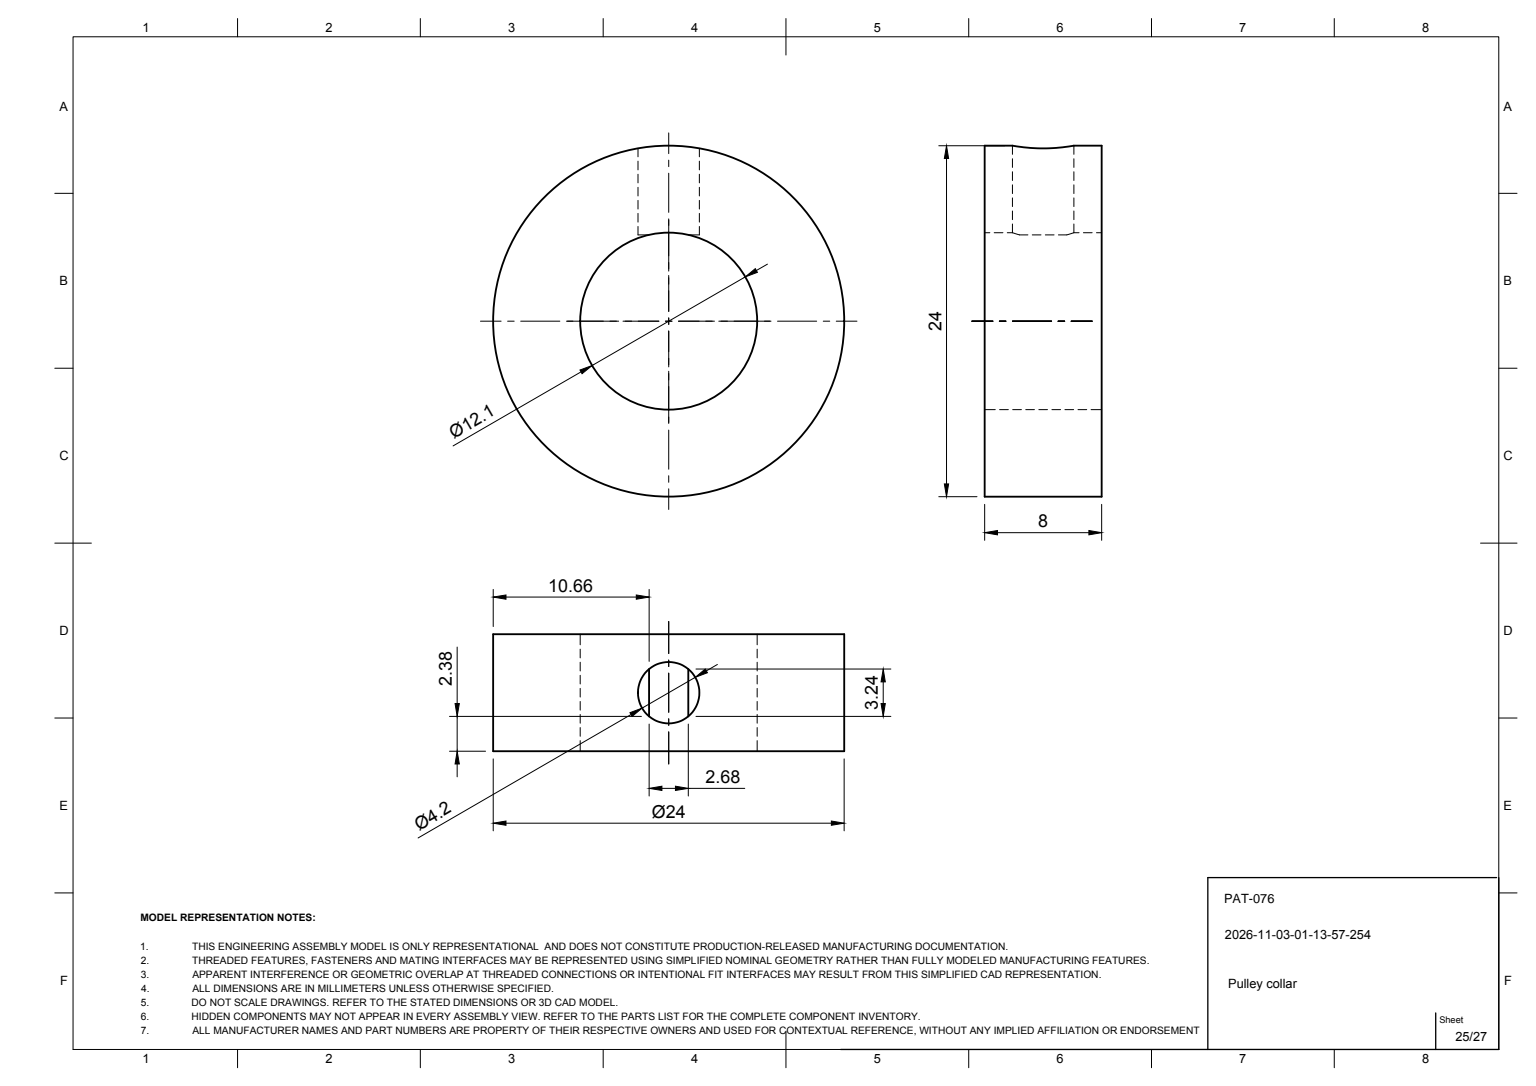
ISO-10303-21;
HEADER;
/* Generated by software containing ST-Developer
 * from STEP Tools, Inc. (www.steptools.com) 
 */

FILE_DESCRIPTION(
/* description */ ('Overhung pulley bearing cartridge'),
/* implementation_level */ '2;1');

FILE_NAME(
/* name */ 'Pulley collar.step',
/* time_stamp */ '2026-10-28T03:22:33-07:00',
/* author */ (''),
/* organization */ (''),
/* preprocessor_version */ 'ST-DEVELOPER v20.2',
/* originating_system */ 'Autodesk Translation Framework v15.17.0.0',
/* authorisation */ '');

FILE_SCHEMA (('AUTOMOTIVE_DESIGN { 1 0 10303 214 3 1 1 }'));
ENDSEC;

DATA;
#10=MECHANICAL_DESIGN_GEOMETRIC_PRESENTATION_REPRESENTATION('',(#309),#10963);
#185=B_SPLINE_CURVE_WITH_KNOTS('',3,(#9899,#9900,#9901,#9902,#9903,#9904,
#9905,#9906,#9907,#9908),.UNSPECIFIED.,.F.,.F.,(4,2,2,2,4),(0.818088904349169,
0.878131747417166,0.957937926194037,1.03774410497091,1.0977869480389),
 .UNSPECIFIED.);
#186=B_SPLINE_CURVE_WITH_KNOTS('',3,(#9914,#9915,#9916,#9917,#9918,#9919,
#9920,#9921,#9922,#9923,#9924,#9925,#9926,#9927,#9928,#9929,#9930,#9931),
 .UNSPECIFIED.,.F.,.F.,(4,2,2,2,2,2,2,2,4),(0.,0.0792812130427884,0.158562426085577,
0.237841058284634,0.317119690483692,0.396398322682749,0.475676954881807,
0.554958167924595,0.634239380967384),.UNSPECIFIED.);
#187=B_SPLINE_CURVE_WITH_KNOTS('',3,(#9932,#9933,#9934,#9935,#9936,#9937,
#9938,#9939,#9940,#9941,#9942,#9943,#9944,#9945,#9946,#9947,#9948,#9949),
 .UNSPECIFIED.,.F.,.F.,(4,2,2,2,2,2,2,2,4),(0.634239380967384,0.713520594010172,
0.792801807052961,0.872080439252018,0.951359071451076,1.03063770365013,
1.10991633584919,1.18919754889198,1.26847876193477),.UNSPECIFIED.);
#188=B_SPLINE_CURVE_WITH_KNOTS('',3,(#9952,#9953,#9954,#9955,#9956,#9957,
#9958,#9959,#9960,#9961),.UNSPECIFIED.,.F.,.F.,(4,2,2,2,4),(0.17946362021981,
0.239506463287808,0.319312642064679,0.39911882084155,0.459161663909547),
 .UNSPECIFIED.);
#257=SHAPE_REPRESENTATION_RELATIONSHIP('SRR','None',#11079,#279);
#279=ADVANCED_BREP_SHAPE_REPRESENTATION('',(#337),#10959);
#309=STYLED_ITEM('',(#11267),#337);
#337=MANIFOLD_SOLID_BREP('Body1',#5678);
#417=FACE_BOUND('',#1190,.T.);
#418=FACE_BOUND('',#1192,.T.);
#419=FACE_BOUND('',#1194,.T.);
#420=FACE_BOUND('',#1196,.T.);
#546=PLANE('',#6370);
#547=PLANE('',#6375);
#548=PLANE('',#6382);
#549=PLANE('',#6383);
#781=FACE_OUTER_BOUND('',#1186,.T.);
#782=FACE_OUTER_BOUND('',#1187,.T.);
#783=FACE_OUTER_BOUND('',#1188,.T.);
#784=FACE_OUTER_BOUND('',#1189,.T.);
#785=FACE_OUTER_BOUND('',#1191,.T.);
#786=FACE_OUTER_BOUND('',#1193,.T.);
#787=FACE_OUTER_BOUND('',#1195,.T.);
#1186=EDGE_LOOP('',(#4467,#4468));
#1187=EDGE_LOOP('',(#4469,#4470,#4471,#4472,#4473,#4474,#4475,#4476,#4477));
#1188=EDGE_LOOP('',(#4478,#4479,#4480));
#1189=EDGE_LOOP('',(#4481,#4482,#4483,#4484));
#1190=EDGE_LOOP('',(#4485,#4486,#4487,#4488));
#1191=EDGE_LOOP('',(#4489,#4490,#4491,#4492));
#1192=EDGE_LOOP('',(#4493,#4494));
#1193=EDGE_LOOP('',(#4495));
#1194=EDGE_LOOP('',(#4496));
#1195=EDGE_LOOP('',(#4497));
#1196=EDGE_LOOP('',(#4498));
#1522=LINE('',#9895,#1864);
#1523=LINE('',#9912,#1865);
#1524=LINE('',#9963,#1866);
#1525=LINE('',#9968,#1867);
#1526=LINE('',#9974,#1868);
#1864=VECTOR('',#7774,1.);
#1865=VECTOR('',#7781,0.21);
#1866=VECTOR('',#7786,1.);
#1867=VECTOR('',#7791,0.605);
#1868=VECTOR('',#7798,1.2);
#2203=CIRCLE('',#6371,0.21);
#2204=CIRCLE('',#6373,0.21);
#2205=CIRCLE('',#6374,0.21);
#2206=CIRCLE('',#6377,0.605);
#2207=CIRCLE('',#6378,0.605);
#2208=CIRCLE('',#6380,1.2);
#2209=CIRCLE('',#6381,1.2);
#2660=VERTEX_POINT('',#9893);
#2661=VERTEX_POINT('',#9894);
#2662=VERTEX_POINT('',#9898);
#2663=VERTEX_POINT('',#9909);
#2664=VERTEX_POINT('',#9911);
#2665=VERTEX_POINT('',#9913);
#2666=VERTEX_POINT('',#9950);
#2667=VERTEX_POINT('',#9965);
#2668=VERTEX_POINT('',#9967);
#2669=VERTEX_POINT('',#9971);
#2670=VERTEX_POINT('',#9973);
#3303=EDGE_CURVE('',#2660,#2661,#1522,.T.);
#3304=EDGE_CURVE('',#2660,#2661,#2203,.T.);
#3305=EDGE_CURVE('',#2662,#2660,#185,.T.);
#3306=EDGE_CURVE('',#2663,#2662,#2204,.T.);
#3307=EDGE_CURVE('',#2663,#2664,#1523,.T.);
#3308=EDGE_CURVE('',#2665,#2664,#186,.T.);
#3309=EDGE_CURVE('',#2664,#2665,#187,.T.);
#3310=EDGE_CURVE('',#2666,#2663,#2205,.T.);
#3311=EDGE_CURVE('',#2661,#2666,#188,.T.);
#3312=EDGE_CURVE('',#2666,#2662,#1524,.T.);
#3313=EDGE_CURVE('',#2667,#2667,#2206,.T.);
#3314=EDGE_CURVE('',#2667,#2668,#1525,.T.);
#3315=EDGE_CURVE('',#2668,#2668,#2207,.T.);
#3316=EDGE_CURVE('',#2669,#2669,#2208,.T.);
#3317=EDGE_CURVE('',#2669,#2670,#1526,.T.);
#3318=EDGE_CURVE('',#2670,#2670,#2209,.T.);
#4467=ORIENTED_EDGE('',*,*,#3303,.F.);
#4468=ORIENTED_EDGE('',*,*,#3304,.T.);
#4469=ORIENTED_EDGE('',*,*,#3305,.F.);
#4470=ORIENTED_EDGE('',*,*,#3306,.F.);
#4471=ORIENTED_EDGE('',*,*,#3307,.T.);
#4472=ORIENTED_EDGE('',*,*,#3308,.F.);
#4473=ORIENTED_EDGE('',*,*,#3309,.F.);
#4474=ORIENTED_EDGE('',*,*,#3307,.F.);
#4475=ORIENTED_EDGE('',*,*,#3310,.F.);
#4476=ORIENTED_EDGE('',*,*,#3311,.F.);
#4477=ORIENTED_EDGE('',*,*,#3304,.F.);
#4478=ORIENTED_EDGE('',*,*,#3312,.F.);
#4479=ORIENTED_EDGE('',*,*,#3310,.T.);
#4480=ORIENTED_EDGE('',*,*,#3306,.T.);
#4481=ORIENTED_EDGE('',*,*,#3313,.F.);
#4482=ORIENTED_EDGE('',*,*,#3314,.T.);
#4483=ORIENTED_EDGE('',*,*,#3315,.T.);
#4484=ORIENTED_EDGE('',*,*,#3314,.F.);
#4485=ORIENTED_EDGE('',*,*,#3311,.T.);
#4486=ORIENTED_EDGE('',*,*,#3312,.T.);
#4487=ORIENTED_EDGE('',*,*,#3305,.T.);
#4488=ORIENTED_EDGE('',*,*,#3303,.T.);
#4489=ORIENTED_EDGE('',*,*,#3316,.F.);
#4490=ORIENTED_EDGE('',*,*,#3317,.T.);
#4491=ORIENTED_EDGE('',*,*,#3318,.T.);
#4492=ORIENTED_EDGE('',*,*,#3317,.F.);
#4493=ORIENTED_EDGE('',*,*,#3308,.T.);
#4494=ORIENTED_EDGE('',*,*,#3309,.T.);
#4495=ORIENTED_EDGE('',*,*,#3316,.T.);
#4496=ORIENTED_EDGE('',*,*,#3313,.T.);
#4497=ORIENTED_EDGE('',*,*,#3318,.F.);
#4498=ORIENTED_EDGE('',*,*,#3315,.F.);
#5229=CYLINDRICAL_SURFACE('',#6372,0.21);
#5230=CYLINDRICAL_SURFACE('',#6376,0.605);
#5231=CYLINDRICAL_SURFACE('',#6379,1.2);
#5525=ADVANCED_FACE('',(#781),#546,.T.);
#5526=ADVANCED_FACE('',(#782),#5229,.F.);
#5527=ADVANCED_FACE('',(#783),#547,.T.);
#5528=ADVANCED_FACE('',(#784,#417),#5230,.F.);
#5529=ADVANCED_FACE('',(#785,#418),#5231,.T.);
#5530=ADVANCED_FACE('',(#786,#419),#548,.T.);
#5531=ADVANCED_FACE('',(#787,#420),#549,.F.);
#5678=CLOSED_SHELL('',(#5525,#5526,#5527,#5528,#5529,#5530,#5531));
#6369=AXIS2_PLACEMENT_3D('',#9891,#7770,#7771);
#6370=AXIS2_PLACEMENT_3D('',#9892,#7772,#7773);
#6371=AXIS2_PLACEMENT_3D('',#9896,#7775,#7776);
#6372=AXIS2_PLACEMENT_3D('',#9897,#7777,#7778);
#6373=AXIS2_PLACEMENT_3D('',#9910,#7779,#7780);
#6374=AXIS2_PLACEMENT_3D('',#9951,#7782,#7783);
#6375=AXIS2_PLACEMENT_3D('',#9962,#7784,#7785);
#6376=AXIS2_PLACEMENT_3D('',#9964,#7787,#7788);
#6377=AXIS2_PLACEMENT_3D('',#9966,#7789,#7790);
#6378=AXIS2_PLACEMENT_3D('',#9969,#7792,#7793);
#6379=AXIS2_PLACEMENT_3D('',#9970,#7794,#7795);
#6380=AXIS2_PLACEMENT_3D('',#9972,#7796,#7797);
#6381=AXIS2_PLACEMENT_3D('',#9975,#7799,#7800);
#6382=AXIS2_PLACEMENT_3D('',#9976,#7801,#7802);
#6383=AXIS2_PLACEMENT_3D('',#9977,#7803,#7804);
#7770=DIRECTION('axis',(0.,0.,1.));
#7771=DIRECTION('refdir',(1.,0.,0.));
#7772=DIRECTION('center_axis',(0.,0.,1.));
#7773=DIRECTION('ref_axis',(1.,0.,0.));
#7774=DIRECTION('',(0.,1.,0.));
#7775=DIRECTION('center_axis',(0.,0.,1.));
#7776=DIRECTION('ref_axis',(1.,0.,0.));
#7777=DIRECTION('center_axis',(0.,0.,1.));
#7778=DIRECTION('ref_axis',(1.,0.,0.));
#7779=DIRECTION('center_axis',(0.,0.,1.));
#7780=DIRECTION('ref_axis',(1.,0.,0.));
#7781=DIRECTION('',(0.,0.,1.));
#7782=DIRECTION('center_axis',(0.,0.,1.));
#7783=DIRECTION('ref_axis',(1.,0.,0.));
#7784=DIRECTION('center_axis',(0.,0.,1.));
#7785=DIRECTION('ref_axis',(1.,0.,0.));
#7786=DIRECTION('',(0.,-1.,0.));
#7787=DIRECTION('center_axis',(0.,1.,0.));
#7788=DIRECTION('ref_axis',(1.,0.,0.));
#7789=DIRECTION('center_axis',(0.,-1.,0.));
#7790=DIRECTION('ref_axis',(1.,0.,0.));
#7791=DIRECTION('',(0.,-1.,0.));
#7792=DIRECTION('center_axis',(0.,-1.,0.));
#7793=DIRECTION('ref_axis',(1.,0.,0.));
#7794=DIRECTION('center_axis',(0.,1.,0.));
#7795=DIRECTION('ref_axis',(1.,0.,0.));
#7796=DIRECTION('center_axis',(0.,1.,0.));
#7797=DIRECTION('ref_axis',(1.,0.,0.));
#7798=DIRECTION('',(0.,-1.,0.));
#7799=DIRECTION('center_axis',(0.,1.,0.));
#7800=DIRECTION('ref_axis',(1.,0.,0.));
#7801=DIRECTION('center_axis',(0.,1.,0.));
#7802=DIRECTION('ref_axis',(1.,0.,0.));
#7803=DIRECTION('center_axis',(0.,1.,0.));
#7804=DIRECTION('ref_axis',(1.,0.,0.));
#9891=CARTESIAN_POINT('',(0.,0.,0.));
#9892=CARTESIAN_POINT('Origin',(0.,10.15,5.09));
#9893=CARTESIAN_POINT('',(0.133884278389959,9.98821310312637,5.09));
#9894=CARTESIAN_POINT('',(0.133884278389959,10.3117868968736,5.09));
#9895=CARTESIAN_POINT('',(0.133884278389959,9.75,5.09));
#9896=CARTESIAN_POINT('Origin',(0.,10.15,5.09));
#9897=CARTESIAN_POINT('Origin',(0.,10.15,5.09));
#9898=CARTESIAN_POINT('',(-0.133884278389959,9.98821310312637,5.09));
#9899=CARTESIAN_POINT('Ctrl Pts',(-0.13388427838996,9.98821310312637,5.09));
#9900=CARTESIAN_POINT('Ctrl Pts',(-0.118254395260805,9.97527883178237,5.09354677224418));
#9901=CARTESIAN_POINT('Ctrl Pts',(-0.1001097876823,9.96420068341256,5.09698224789957));
#9902=CARTESIAN_POINT('Ctrl Pts',(-0.054829872132519,9.94536143894557,5.1030741628997));
#9903=CARTESIAN_POINT('Ctrl Pts',(-0.0266020595922903,9.94,5.105));
#9904=CARTESIAN_POINT('Ctrl Pts',(0.0266020595922903,9.94,5.105));
#9905=CARTESIAN_POINT('Ctrl Pts',(0.0548298721325189,9.94536143894557,5.1030741628997));
#9906=CARTESIAN_POINT('Ctrl Pts',(0.1001097876823,9.96420068341256,5.09698224789957));
#9907=CARTESIAN_POINT('Ctrl Pts',(0.118254395260804,9.97527883178237,5.09354677224418));
#9908=CARTESIAN_POINT('Ctrl Pts',(0.133884278389959,9.98821310312637,5.09));
#9909=CARTESIAN_POINT('',(-0.21,10.15,5.09));
#9910=CARTESIAN_POINT('Origin',(0.,10.15,5.09));
#9911=CARTESIAN_POINT('',(-0.21,10.15,5.68148212005091));
#9912=CARTESIAN_POINT('',(-0.21,10.15,5.09));
#9913=CARTESIAN_POINT('',(0.21,10.15,5.68148212005091));
#9914=CARTESIAN_POINT('Ctrl Pts',(0.21,10.15,5.68148212005091));
#9915=CARTESIAN_POINT('Ctrl Pts',(0.21,10.1235729289857,5.68148212005091));
#9916=CARTESIAN_POINT('Ctrl Pts',(0.204707379175836,10.0954224459113,5.68246056146672));
#9917=CARTESIAN_POINT('Ctrl Pts',(0.183259409780014,10.0436994304444,5.68597389417424));
#9918=CARTESIAN_POINT('Ctrl Pts',(0.167106958412512,10.0201221103142,5.68845578531258));
#9919=CARTESIAN_POINT('Ctrl Pts',(0.129878495645339,9.98289364754699,5.6930982535617));
#9920=CARTESIAN_POINT('Ctrl Pts',(0.106300916040875,9.96674072098398,5.69556345497295));
#9921=CARTESIAN_POINT('Ctrl Pts',(0.0545770066794469,9.94529240674315,5.69903845223025));
#9922=CARTESIAN_POINT('Ctrl Pts',(0.0264262107330192,9.94,5.7));
#9923=CARTESIAN_POINT('Ctrl Pts',(-0.0264262107330192,9.94,5.7));
#9924=CARTESIAN_POINT('Ctrl Pts',(-0.0545770066794469,9.94529240674315,
5.69903845223025));
#9925=CARTESIAN_POINT('Ctrl Pts',(-0.106300916040875,9.96674072098398,5.69556345497295));
#9926=CARTESIAN_POINT('Ctrl Pts',(-0.129878495645339,9.98289364754699,5.6930982535617));
#9927=CARTESIAN_POINT('Ctrl Pts',(-0.167106958412512,10.0201221103142,5.68845578531258));
#9928=CARTESIAN_POINT('Ctrl Pts',(-0.183259409780014,10.0436994304444,5.68597389417424));
#9929=CARTESIAN_POINT('Ctrl Pts',(-0.204707379175836,10.0954224459113,5.68246056146672));
#9930=CARTESIAN_POINT('Ctrl Pts',(-0.21,10.1235729289857,5.68148212005091));
#9931=CARTESIAN_POINT('Ctrl Pts',(-0.21,10.15,5.68148212005091));
#9932=CARTESIAN_POINT('Ctrl Pts',(-0.21,10.15,5.68148212005091));
#9933=CARTESIAN_POINT('Ctrl Pts',(-0.21,10.1764270710143,5.68148212005091));
#9934=CARTESIAN_POINT('Ctrl Pts',(-0.204707379175836,10.2045775540887,5.68246056146672));
#9935=CARTESIAN_POINT('Ctrl Pts',(-0.183259409780014,10.2563005695556,5.68597389417424));
#9936=CARTESIAN_POINT('Ctrl Pts',(-0.167106958412512,10.2798778896858,5.68845578531258));
#9937=CARTESIAN_POINT('Ctrl Pts',(-0.129878495645339,10.317106352453,5.6930982535617));
#9938=CARTESIAN_POINT('Ctrl Pts',(-0.106300916040875,10.333259279016,5.69556345497295));
#9939=CARTESIAN_POINT('Ctrl Pts',(-0.0545770066794469,10.3547075932569,
5.69903845223025));
#9940=CARTESIAN_POINT('Ctrl Pts',(-0.0264262107330192,10.36,5.7));
#9941=CARTESIAN_POINT('Ctrl Pts',(0.0264262107330191,10.36,5.7));
#9942=CARTESIAN_POINT('Ctrl Pts',(0.0545770066794468,10.3547075932569,5.69903845223025));
#9943=CARTESIAN_POINT('Ctrl Pts',(0.106300916040875,10.333259279016,5.69556345497295));
#9944=CARTESIAN_POINT('Ctrl Pts',(0.129878495645339,10.317106352453,5.6930982535617));
#9945=CARTESIAN_POINT('Ctrl Pts',(0.167106958412512,10.2798778896858,5.68845578531258));
#9946=CARTESIAN_POINT('Ctrl Pts',(0.183259409780014,10.2563005695556,5.68597389417424));
#9947=CARTESIAN_POINT('Ctrl Pts',(0.204707379175836,10.2045775540887,5.68246056146672));
#9948=CARTESIAN_POINT('Ctrl Pts',(0.21,10.1764270710143,5.68148212005091));
#9949=CARTESIAN_POINT('Ctrl Pts',(0.21,10.15,5.68148212005091));
#9950=CARTESIAN_POINT('',(-0.133884278389959,10.3117868968736,5.09));
#9951=CARTESIAN_POINT('Origin',(0.,10.15,5.09));
#9952=CARTESIAN_POINT('Ctrl Pts',(0.13388427838996,10.3117868968736,5.09));
#9953=CARTESIAN_POINT('Ctrl Pts',(0.118254395260805,10.3247211682176,5.09354677224418));
#9954=CARTESIAN_POINT('Ctrl Pts',(0.1001097876823,10.3357993165874,5.09698224789957));
#9955=CARTESIAN_POINT('Ctrl Pts',(0.054829872132519,10.3546385610544,5.1030741628997));
#9956=CARTESIAN_POINT('Ctrl Pts',(0.0266020595922903,10.36,5.105));
#9957=CARTESIAN_POINT('Ctrl Pts',(-0.0266020595922903,10.36,5.105));
#9958=CARTESIAN_POINT('Ctrl Pts',(-0.0548298721325189,10.3546385610544,
5.1030741628997));
#9959=CARTESIAN_POINT('Ctrl Pts',(-0.1001097876823,10.3357993165874,5.09698224789957));
#9960=CARTESIAN_POINT('Ctrl Pts',(-0.118254395260804,10.3247211682176,5.09354677224418));
#9961=CARTESIAN_POINT('Ctrl Pts',(-0.133884278389959,10.3117868968736,5.09));
#9962=CARTESIAN_POINT('Origin',(0.,10.15,5.09));
#9963=CARTESIAN_POINT('',(-0.133884278389959,9.75,5.09));
#9964=CARTESIAN_POINT('Origin',(0.,9.75,4.5));
#9965=CARTESIAN_POINT('',(-0.605,10.55,4.5));
#9966=CARTESIAN_POINT('Origin',(0.,10.55,4.5));
#9967=CARTESIAN_POINT('',(-0.605,9.75,4.5));
#9968=CARTESIAN_POINT('',(-0.605,9.75,4.5));
#9969=CARTESIAN_POINT('Origin',(0.,9.75,4.5));
#9970=CARTESIAN_POINT('Origin',(0.,9.75,4.5));
#9971=CARTESIAN_POINT('',(-1.2,10.55,4.5));
#9972=CARTESIAN_POINT('Origin',(0.,10.55,4.5));
#9973=CARTESIAN_POINT('',(-1.2,9.75,4.5));
#9974=CARTESIAN_POINT('',(-1.2,9.75,4.5));
#9975=CARTESIAN_POINT('Origin',(0.,9.75,4.5));
#9976=CARTESIAN_POINT('Origin',(0.,10.55,4.5));
#9977=CARTESIAN_POINT('Origin',(0.,9.75,4.5));
#10932=UNCERTAINTY_MEASURE_WITH_UNIT(LENGTH_MEASURE(0.001),#10964,
'DISTANCE_ACCURACY_VALUE',
'Maximum model space distance between geometric entities at asserted c
onnectivities');
#10936=UNCERTAINTY_MEASURE_WITH_UNIT(LENGTH_MEASURE(0.001),#10964,
'DISTANCE_ACCURACY_VALUE',
'Maximum model space distance between geometric entities at asserted c
onnectivities');
#10959=(
GEOMETRIC_REPRESENTATION_CONTEXT(3)
GLOBAL_UNCERTAINTY_ASSIGNED_CONTEXT((#10932))
GLOBAL_UNIT_ASSIGNED_CONTEXT((#10964,#10966,#10967))
REPRESENTATION_CONTEXT('','3D')
);
#10963=(
GEOMETRIC_REPRESENTATION_CONTEXT(3)
GLOBAL_UNCERTAINTY_ASSIGNED_CONTEXT((#10936))
GLOBAL_UNIT_ASSIGNED_CONTEXT((#10964,#10966,#10967))
REPRESENTATION_CONTEXT('','3D')
);
#10964=(
LENGTH_UNIT()
NAMED_UNIT(*)
SI_UNIT(.CENTI.,.METRE.)
);
#10966=(
NAMED_UNIT(*)
PLANE_ANGLE_UNIT()
SI_UNIT($,.RADIAN.)
);
#10967=(
NAMED_UNIT(*)
SI_UNIT($,.STERADIAN.)
SOLID_ANGLE_UNIT()
);
#10990=SHAPE_DEFINITION_REPRESENTATION(#11043,#11079);
#11043=PRODUCT_DEFINITION_SHAPE('',$,#11106);
#11079=SHAPE_REPRESENTATION('',(#6369),#10959);
#11083=PRODUCT_DEFINITION_CONTEXT('part definition',#11163,'design');
#11106=PRODUCT_DEFINITION('Pulley collar','Pulley collar',#11132,#11083);
#11132=PRODUCT_DEFINITION_FORMATION('',$,#11187);
#11163=APPLICATION_CONTEXT(
'Core Data for Automotive Mechanical Design Process');
#11164=PRODUCT_CONTEXT('part definition',#11163,'mechanical');
#11187=PRODUCT('Pulley collar','Pulley collar','Pulley collar',(#11164));
#11261=COLOUR_RGB('Off White',0.89,0.88,0.83);
#11262=FILL_AREA_STYLE_COLOUR('',#11261);
#11263=FILL_AREA_STYLE('',(#11262));
#11264=SURFACE_STYLE_FILL_AREA(#11263);
#11265=SURFACE_SIDE_STYLE('',(#11264));
#11266=SURFACE_STYLE_USAGE(.BOTH.,#11265);
#11267=PRESENTATION_STYLE_ASSIGNMENT((#11266));
ENDSEC;
END-ISO-10303-21;
